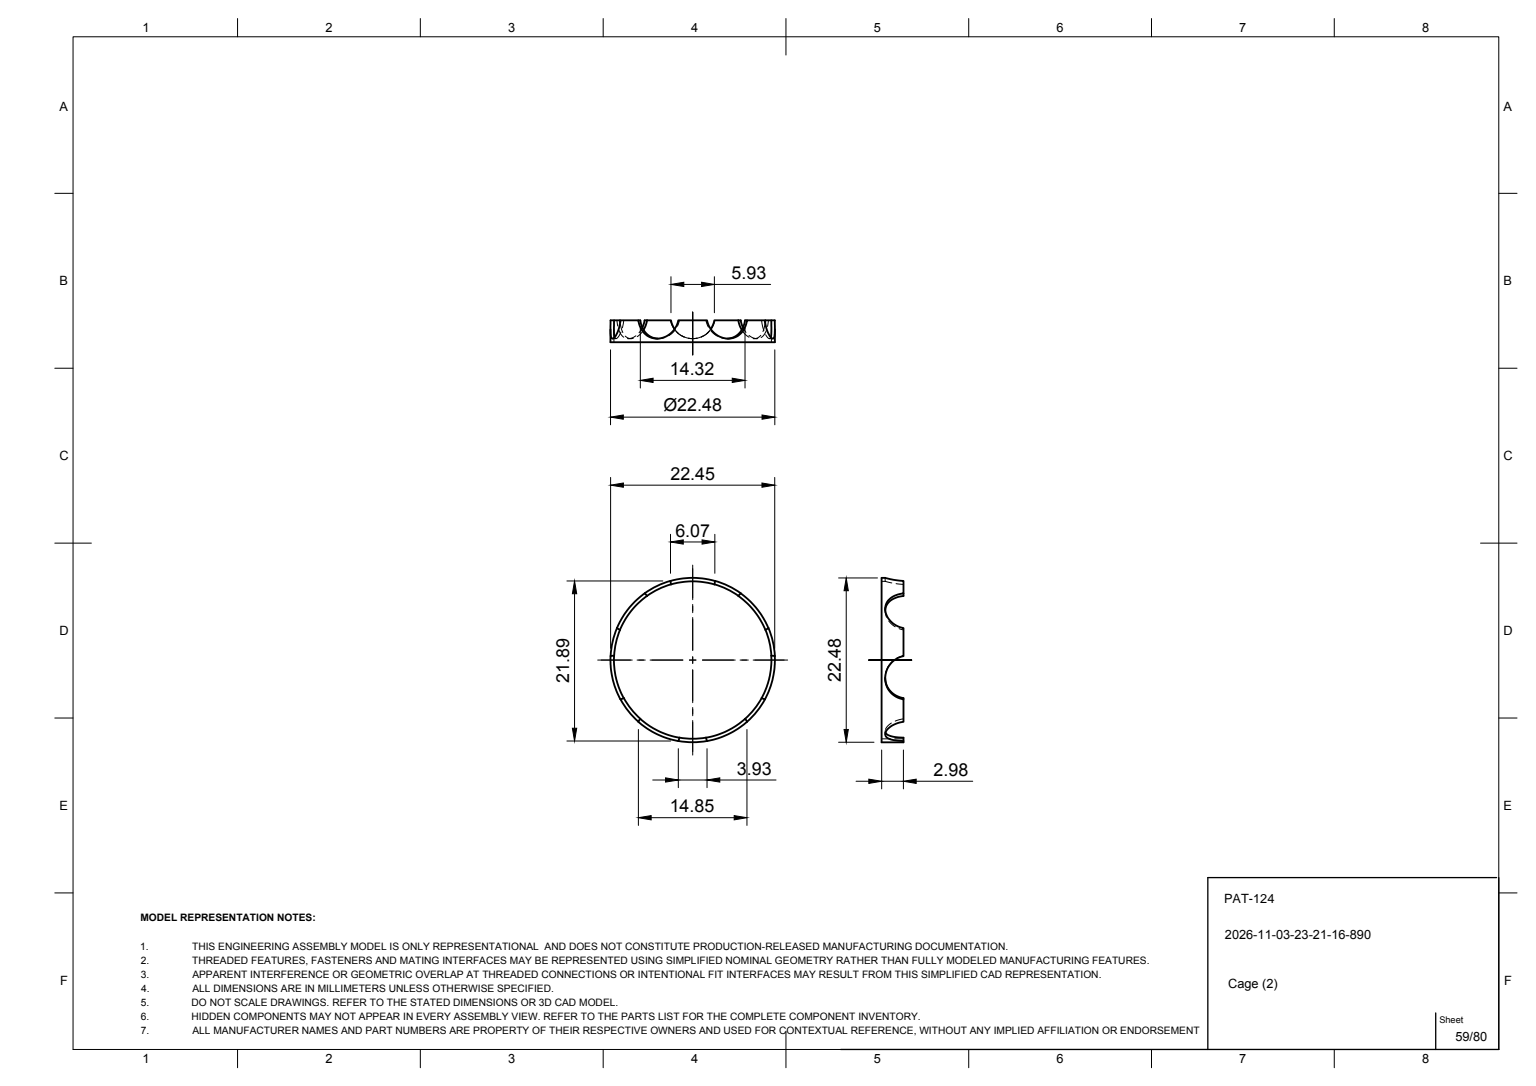
ISO-10303-21;
HEADER;
/* Generated by software containing ST-Developer
 * from STEP Tools, Inc. (www.steptools.com) 
 */

FILE_DESCRIPTION(
/* description */ ('XY cross-slide table'),
/* implementation_level */ '2;1');

FILE_NAME(
/* name */ 'Cage (2).step',
/* time_stamp */ '2026-10-28T03:22:46-07:00',
/* author */ (''),
/* organization */ (''),
/* preprocessor_version */ 'ST-DEVELOPER v20.2',
/* originating_system */ 'Autodesk Translation Framework v15.17.0.0',
/* authorisation */ '');

FILE_SCHEMA (('AUTOMOTIVE_DESIGN { 1 0 10303 214 3 1 1 }'));
ENDSEC;

DATA;
#10=MECHANICAL_DESIGN_GEOMETRIC_PRESENTATION_REPRESENTATION('',(#1745),#62984);
#1037=B_SPLINE_CURVE_WITH_KNOTS('',3,(#48636,#48637,#48638,#48639,#48640,
#48641,#48642,#48643,#48644,#48645,#48646,#48647,#48648,#48649,#48650,#48651,
#48652,#48653,#48654,#48655,#48656,#48657),.UNSPECIFIED.,.F.,.F.,(4,2,2,
2,2,2,2,2,2,2,4),(0.0591825211272536,0.157966726598481,0.236950089897721,
0.315933453196962,0.391576304923761,0.46721915665056,0.54286200837736,0.618504860104159,
0.697488223403399,0.77647158670264,0.875255792173867),.UNSPECIFIED.);
#1038=B_SPLINE_CURVE_WITH_KNOTS('',3,(#48661,#48662,#48663,#48664,#48665,
#48666,#48667,#48668,#48669,#48670,#48671,#48672,#48673,#48674,#48675,#48676,
#48677,#48678,#48679,#48680,#48681,#48682),.UNSPECIFIED.,.F.,.F.,(4,2,2,
2,2,2,2,2,2,2,4),(0.0581119756758434,0.106553146291161,0.213106292582322,
0.30849933801665,0.386091982889075,0.4636846277615,0.541277272633925,0.61886991750635,
0.714262962940678,0.820816109231839,0.869257279847157),.UNSPECIFIED.);
#1039=B_SPLINE_CURVE_WITH_KNOTS('',3,(#48688,#48689,#48690,#48691,#48692,
#48693,#48694,#48695,#48696,#48697,#48698,#48699,#48700,#48701,#48702,#48703,
#48704,#48705,#48706,#48707,#48708,#48709),.UNSPECIFIED.,.F.,.F.,(4,2,2,
2,2,2,2,2,2,2,4),(0.0581119756758434,0.106553146291161,0.213106292582322,
0.30849933801665,0.386091982889075,0.4636846277615,0.541277272633925,0.61886991750635,
0.714262962940679,0.820816109231839,0.869257279847157),.UNSPECIFIED.);
#1040=B_SPLINE_CURVE_WITH_KNOTS('',3,(#48713,#48714,#48715,#48716,#48717,
#48718,#48719,#48720,#48721,#48722,#48723,#48724,#48725,#48726,#48727,#48728,
#48729,#48730,#48731,#48732,#48733,#48734),.UNSPECIFIED.,.F.,.F.,(4,2,2,
2,2,2,2,2,2,2,4),(0.0581119756758433,0.106553146291161,0.213106292582322,
0.308499338016649,0.386091982889075,0.4636846277615,0.541277272633925,0.61886991750635,
0.714262962940678,0.820816109231839,0.869257279847157),.UNSPECIFIED.);
#1041=B_SPLINE_CURVE_WITH_KNOTS('',3,(#48743,#48744,#48745,#48746,#48747,
#48748,#48749,#48750,#48751,#48752,#48753,#48754,#48755,#48756,#48757,#48758,
#48759,#48760,#48761,#48762,#48763,#48764),.UNSPECIFIED.,.F.,.F.,(4,2,2,
2,2,2,2,2,2,2,4),(0.0581119756758433,0.106553146291161,0.213106292582322,
0.30849933801665,0.386091982889075,0.4636846277615,0.541277272633925,0.61886991750635,
0.714262962940678,0.820816109231839,0.869257279847157),.UNSPECIFIED.);
#1042=B_SPLINE_CURVE_WITH_KNOTS('',3,(#48768,#48769,#48770,#48771,#48772,
#48773,#48774,#48775,#48776,#48777,#48778,#48779,#48780,#48781,#48782,#48783,
#48784,#48785,#48786,#48787,#48788,#48789),.UNSPECIFIED.,.F.,.F.,(4,2,2,
2,2,2,2,2,2,2,4),(0.0581119756758434,0.106553146291161,0.213106292582322,
0.30849933801665,0.386091982889075,0.4636846277615,0.541277272633925,0.61886991750635,
0.714262962940678,0.820816109231839,0.869257279847157),.UNSPECIFIED.);
#1043=B_SPLINE_CURVE_WITH_KNOTS('',3,(#48793,#48794,#48795,#48796,#48797,
#48798,#48799,#48800,#48801,#48802,#48803,#48804,#48805,#48806,#48807,#48808,
#48809,#48810,#48811,#48812,#48813,#48814),.UNSPECIFIED.,.F.,.F.,(4,2,2,
2,2,2,2,2,2,2,4),(0.0581119756758434,0.106553146291161,0.213106292582322,
0.30849933801665,0.386091982889075,0.4636846277615,0.541277272633925,0.61886991750635,
0.714262962940678,0.820816109231839,0.869257279847157),.UNSPECIFIED.);
#1044=B_SPLINE_CURVE_WITH_KNOTS('',3,(#48818,#48819,#48820,#48821,#48822,
#48823,#48824,#48825,#48826,#48827,#48828,#48829,#48830,#48831,#48832,#48833,
#48834,#48835,#48836,#48837,#48838,#48839),.UNSPECIFIED.,.F.,.F.,(4,2,2,
2,2,2,2,2,2,2,4),(0.0581119756758433,0.106553146291161,0.213106292582322,
0.30849933801665,0.386091982889075,0.4636846277615,0.541277272633925,0.61886991750635,
0.714262962940678,0.820816109231839,0.869257279847157),.UNSPECIFIED.);
#1045=B_SPLINE_CURVE_WITH_KNOTS('',3,(#48847,#48848,#48849,#48850,#48851,
#48852,#48853,#48854,#48855,#48856,#48857,#48858,#48859,#48860,#48861,#48862,
#48863,#48864,#48865,#48866,#48867,#48868),.UNSPECIFIED.,.F.,.F.,(4,2,2,
2,2,2,2,2,2,2,4),(0.0591825211272536,0.157966726598481,0.236950089897721,
0.315933453196962,0.391576304923761,0.467219156650561,0.54286200837736,
0.618504860104159,0.697488223403399,0.77647158670264,0.875255792173867),
 .UNSPECIFIED.);
#1046=B_SPLINE_CURVE_WITH_KNOTS('',3,(#48876,#48877,#48878,#48879,#48880,
#48881,#48882,#48883,#48884,#48885,#48886,#48887,#48888,#48889,#48890,#48891,
#48892,#48893,#48894,#48895,#48896,#48897),.UNSPECIFIED.,.F.,.F.,(4,2,2,
2,2,2,2,2,2,2,4),(0.0591825211272536,0.157966726598481,0.236950089897722,
0.315933453196962,0.391576304923761,0.467219156650561,0.54286200837736,
0.618504860104159,0.697488223403399,0.77647158670264,0.875255792173867),
 .UNSPECIFIED.);
#1047=B_SPLINE_CURVE_WITH_KNOTS('',3,(#48907,#48908,#48909,#48910,#48911,
#48912,#48913,#48914,#48915,#48916,#48917,#48918,#48919,#48920,#48921,#48922,
#48923,#48924,#48925,#48926,#48927,#48928),.UNSPECIFIED.,.F.,.F.,(4,2,2,
2,2,2,2,2,2,2,4),(0.0591825211272536,0.157966726598481,0.236950089897721,
0.315933453196962,0.391576304923761,0.46721915665056,0.54286200837736,0.618504860104159,
0.697488223403399,0.77647158670264,0.875255792173867),.UNSPECIFIED.);
#1048=B_SPLINE_CURVE_WITH_KNOTS('',3,(#48936,#48937,#48938,#48939,#48940,
#48941,#48942,#48943,#48944,#48945,#48946,#48947,#48948,#48949,#48950,#48951,
#48952,#48953,#48954,#48955,#48956,#48957),.UNSPECIFIED.,.F.,.F.,(4,2,2,
2,2,2,2,2,2,2,4),(0.0591825211272536,0.157966726598481,0.236950089897721,
0.315933453196962,0.391576304923761,0.46721915665056,0.542862008377359,
0.618504860104159,0.697488223403399,0.776471586702639,0.875255792173867),
 .UNSPECIFIED.);
#1049=B_SPLINE_CURVE_WITH_KNOTS('',3,(#48965,#48966,#48967,#48968,#48969,
#48970,#48971,#48972,#48973,#48974,#48975,#48976,#48977,#48978,#48979,#48980,
#48981,#48982,#48983,#48984,#48985,#48986),.UNSPECIFIED.,.F.,.F.,(4,2,2,
2,2,2,2,2,2,2,4),(0.0591825211272536,0.157966726598481,0.236950089897721,
0.315933453196962,0.391576304923761,0.46721915665056,0.54286200837736,0.618504860104159,
0.697488223403399,0.77647158670264,0.875255792173867),.UNSPECIFIED.);
#1050=B_SPLINE_CURVE_WITH_KNOTS('',3,(#48995,#48996,#48997,#48998,#48999,
#49000,#49001,#49002,#49003,#49004,#49005,#49006,#49007,#49008,#49009,#49010,
#49011,#49012,#49013,#49014,#49015,#49016),.UNSPECIFIED.,.F.,.F.,(4,2,2,
2,2,2,2,2,2,2,4),(0.0591825211272536,0.157966726598481,0.236950089897721,
0.315933453196962,0.391576304923761,0.46721915665056,0.542862008377359,
0.618504860104159,0.697488223403399,0.776471586702639,0.875255792173867),
 .UNSPECIFIED.);
#1418=SPHERICAL_SURFACE('',#25587,0.309556);
#1419=SPHERICAL_SURFACE('',#25603,0.309556);
#1420=SPHERICAL_SURFACE('',#25608,0.309556);
#1421=SPHERICAL_SURFACE('',#25614,0.309556);
#1422=SPHERICAL_SURFACE('',#25619,0.309556);
#1423=SPHERICAL_SURFACE('',#25624,0.309556);
#1424=SPHERICAL_SURFACE('',#25632,0.309556);
#1558=SHAPE_REPRESENTATION_RELATIONSHIP('SRR','None',#63414,#1641);
#1641=ADVANCED_BREP_SHAPE_REPRESENTATION('',(#1854),#62951);
#1745=STYLED_ITEM('',(#63912),#1854);
#1854=MANIFOLD_SOLID_BREP('Continuous crown cage',#23043);
#2205=FACE_BOUND('',#5346,.T.);
#2666=PLANE('',#25600);
#2667=PLANE('',#25605);
#2668=PLANE('',#25610);
#2669=PLANE('',#25616);
#2670=PLANE('',#25621);
#2671=PLANE('',#25630);
#2672=PLANE('',#25634);
#2673=PLANE('',#25635);
#3698=FACE_OUTER_BOUND('',#5330,.T.);
#3699=FACE_OUTER_BOUND('',#5331,.T.);
#3700=FACE_OUTER_BOUND('',#5332,.T.);
#3701=FACE_OUTER_BOUND('',#5333,.T.);
#3702=FACE_OUTER_BOUND('',#5334,.T.);
#3703=FACE_OUTER_BOUND('',#5335,.T.);
#3704=FACE_OUTER_BOUND('',#5336,.T.);
#3705=FACE_OUTER_BOUND('',#5337,.T.);
#3706=FACE_OUTER_BOUND('',#5338,.T.);
#3707=FACE_OUTER_BOUND('',#5339,.T.);
#3708=FACE_OUTER_BOUND('',#5340,.T.);
#3709=FACE_OUTER_BOUND('',#5341,.T.);
#3710=FACE_OUTER_BOUND('',#5342,.T.);
#3711=FACE_OUTER_BOUND('',#5343,.T.);
#3712=FACE_OUTER_BOUND('',#5344,.T.);
#3713=FACE_OUTER_BOUND('',#5345,.T.);
#3714=FACE_OUTER_BOUND('',#5347,.T.);
#5330=EDGE_LOOP('',(#18706,#18707,#18708,#18709));
#5331=EDGE_LOOP('',(#18710,#18711,#18712,#18713,#18714,#18715,#18716,#18717,
#18718,#18719,#18720,#18721,#18722,#18723,#18724,#18725,#18726,#18727));
#5332=EDGE_LOOP('',(#18728,#18729,#18730,#18731));
#5333=EDGE_LOOP('',(#18732,#18733,#18734,#18735));
#5334=EDGE_LOOP('',(#18736,#18737,#18738,#18739));
#5335=EDGE_LOOP('',(#18740,#18741,#18742,#18743));
#5336=EDGE_LOOP('',(#18744,#18745,#18746,#18747,#18748,#18749));
#5337=EDGE_LOOP('',(#18750,#18751,#18752,#18753));
#5338=EDGE_LOOP('',(#18754,#18755,#18756,#18757));
#5339=EDGE_LOOP('',(#18758,#18759,#18760,#18761));
#5340=EDGE_LOOP('',(#18762,#18763,#18764,#18765));
#5341=EDGE_LOOP('',(#18766,#18767,#18768,#18769));
#5342=EDGE_LOOP('',(#18770,#18771,#18772,#18773,#18774,#18775,#18776,#18777,
#18778,#18779,#18780,#18781,#18782,#18783,#18784,#18785,#18786,#18787));
#5343=EDGE_LOOP('',(#18788,#18789,#18790,#18791));
#5344=EDGE_LOOP('',(#18792,#18793,#18794,#18795));
#5345=EDGE_LOOP('',(#18796));
#5346=EDGE_LOOP('',(#18797));
#5347=EDGE_LOOP('',(#18798,#18799,#18800,#18801));
#6847=LINE('',#48738,#8334);
#6848=LINE('',#48991,#8335);
#8334=VECTOR('',#30590,1.123812);
#8335=VECTOR('',#30659,1.076188);
#9496=CIRCLE('',#25588,0.303778037777585);
#9497=CIRCLE('',#25589,0.303778037777585);
#9498=CIRCLE('',#25591,1.123812);
#9499=CIRCLE('',#25592,1.123812);
#9500=CIRCLE('',#25593,1.123812);
#9501=CIRCLE('',#25594,1.123812);
#9502=CIRCLE('',#25595,1.123812);
#9503=CIRCLE('',#25596,1.123812);
#9504=CIRCLE('',#25597,1.123812);
#9505=CIRCLE('',#25598,1.123812);
#9506=CIRCLE('',#25599,1.123812);
#9507=CIRCLE('',#25601,1.076188);
#9508=CIRCLE('',#25602,0.303778037777585);
#9509=CIRCLE('',#25604,0.303778037777585);
#9510=CIRCLE('',#25606,1.076188);
#9511=CIRCLE('',#25607,0.303778037777585);
#9512=CIRCLE('',#25609,0.303778037777585);
#9513=CIRCLE('',#25611,1.076188);
#9514=CIRCLE('',#25612,1.076188);
#9515=CIRCLE('',#25613,0.303778037777585);
#9516=CIRCLE('',#25615,0.303778037777585);
#9517=CIRCLE('',#25617,1.076188);
#9518=CIRCLE('',#25618,0.303778037777585);
#9519=CIRCLE('',#25620,0.303778037777585);
#9520=CIRCLE('',#25622,1.076188);
#9521=CIRCLE('',#25623,0.303778037777585);
#9522=CIRCLE('',#25625,0.303778037777585);
#9523=CIRCLE('',#25627,1.076188);
#9524=CIRCLE('',#25628,1.076188);
#9525=CIRCLE('',#25629,1.076188);
#9526=CIRCLE('',#25631,0.303778037777585);
#9527=CIRCLE('',#25633,0.303778037777585);
#11055=VERTEX_POINT('',#48634);
#11056=VERTEX_POINT('',#48635);
#11057=VERTEX_POINT('',#48658);
#11058=VERTEX_POINT('',#48660);
#11059=VERTEX_POINT('',#48685);
#11060=VERTEX_POINT('',#48687);
#11061=VERTEX_POINT('',#48710);
#11062=VERTEX_POINT('',#48712);
#11063=VERTEX_POINT('',#48735);
#11064=VERTEX_POINT('',#48737);
#11065=VERTEX_POINT('',#48740);
#11066=VERTEX_POINT('',#48742);
#11067=VERTEX_POINT('',#48765);
#11068=VERTEX_POINT('',#48767);
#11069=VERTEX_POINT('',#48790);
#11070=VERTEX_POINT('',#48792);
#11071=VERTEX_POINT('',#48815);
#11072=VERTEX_POINT('',#48817);
#11073=VERTEX_POINT('',#48842);
#11074=VERTEX_POINT('',#48846);
#11075=VERTEX_POINT('',#48871);
#11076=VERTEX_POINT('',#48875);
#11077=VERTEX_POINT('',#48900);
#11078=VERTEX_POINT('',#48902);
#11079=VERTEX_POINT('',#48906);
#11080=VERTEX_POINT('',#48931);
#11081=VERTEX_POINT('',#48935);
#11082=VERTEX_POINT('',#48960);
#11083=VERTEX_POINT('',#48964);
#11084=VERTEX_POINT('',#48989);
#11085=VERTEX_POINT('',#48992);
#11086=VERTEX_POINT('',#48994);
#13737=EDGE_CURVE('',#11055,#11056,#1037,.T.);
#13738=EDGE_CURVE('',#11057,#11055,#9496,.T.);
#13739=EDGE_CURVE('',#11058,#11057,#1038,.T.);
#13740=EDGE_CURVE('',#11056,#11058,#9497,.T.);
#13741=EDGE_CURVE('',#11059,#11057,#9498,.T.);
#13742=EDGE_CURVE('',#11059,#11060,#1039,.T.);
#13743=EDGE_CURVE('',#11061,#11060,#9499,.T.);
#13744=EDGE_CURVE('',#11061,#11062,#1040,.T.);
#13745=EDGE_CURVE('',#11063,#11062,#9500,.T.);
#13746=EDGE_CURVE('',#11063,#11064,#6847,.T.);
#13747=EDGE_CURVE('',#11064,#11064,#9501,.T.);
#13748=EDGE_CURVE('',#11065,#11063,#9502,.T.);
#13749=EDGE_CURVE('',#11065,#11066,#1041,.T.);
#13750=EDGE_CURVE('',#11067,#11066,#9503,.T.);
#13751=EDGE_CURVE('',#11067,#11068,#1042,.T.);
#13752=EDGE_CURVE('',#11069,#11068,#9504,.T.);
#13753=EDGE_CURVE('',#11069,#11070,#1043,.T.);
#13754=EDGE_CURVE('',#11071,#11070,#9505,.T.);
#13755=EDGE_CURVE('',#11071,#11072,#1044,.T.);
#13756=EDGE_CURVE('',#11058,#11072,#9506,.T.);
#13757=EDGE_CURVE('',#11055,#11073,#9507,.T.);
#13758=EDGE_CURVE('',#11073,#11059,#9508,.T.);
#13759=EDGE_CURVE('',#11074,#11073,#1045,.T.);
#13760=EDGE_CURVE('',#11060,#11074,#9509,.T.);
#13761=EDGE_CURVE('',#11074,#11075,#9510,.T.);
#13762=EDGE_CURVE('',#11075,#11061,#9511,.T.);
#13763=EDGE_CURVE('',#11076,#11075,#1046,.T.);
#13764=EDGE_CURVE('',#11062,#11076,#9512,.T.);
#13765=EDGE_CURVE('',#11076,#11077,#9513,.T.);
#13766=EDGE_CURVE('',#11077,#11078,#9514,.T.);
#13767=EDGE_CURVE('',#11078,#11065,#9515,.T.);
#13768=EDGE_CURVE('',#11079,#11078,#1047,.T.);
#13769=EDGE_CURVE('',#11066,#11079,#9516,.T.);
#13770=EDGE_CURVE('',#11079,#11080,#9517,.T.);
#13771=EDGE_CURVE('',#11080,#11067,#9518,.T.);
#13772=EDGE_CURVE('',#11081,#11080,#1048,.T.);
#13773=EDGE_CURVE('',#11068,#11081,#9519,.T.);
#13774=EDGE_CURVE('',#11081,#11082,#9520,.T.);
#13775=EDGE_CURVE('',#11082,#11069,#9521,.T.);
#13776=EDGE_CURVE('',#11083,#11082,#1049,.T.);
#13777=EDGE_CURVE('',#11070,#11083,#9522,.T.);
#13778=EDGE_CURVE('',#11084,#11084,#9523,.T.);
#13779=EDGE_CURVE('',#11084,#11077,#6848,.T.);
#13780=EDGE_CURVE('',#11085,#11056,#9524,.T.);
#13781=EDGE_CURVE('',#11085,#11086,#1050,.T.);
#13782=EDGE_CURVE('',#11083,#11086,#9525,.T.);
#13783=EDGE_CURVE('',#11072,#11085,#9526,.T.);
#13784=EDGE_CURVE('',#11086,#11071,#9527,.T.);
#18706=ORIENTED_EDGE('',*,*,#13737,.F.);
#18707=ORIENTED_EDGE('',*,*,#13738,.F.);
#18708=ORIENTED_EDGE('',*,*,#13739,.F.);
#18709=ORIENTED_EDGE('',*,*,#13740,.F.);
#18710=ORIENTED_EDGE('',*,*,#13739,.T.);
#18711=ORIENTED_EDGE('',*,*,#13741,.F.);
#18712=ORIENTED_EDGE('',*,*,#13742,.T.);
#18713=ORIENTED_EDGE('',*,*,#13743,.F.);
#18714=ORIENTED_EDGE('',*,*,#13744,.T.);
#18715=ORIENTED_EDGE('',*,*,#13745,.F.);
#18716=ORIENTED_EDGE('',*,*,#13746,.T.);
#18717=ORIENTED_EDGE('',*,*,#13747,.F.);
#18718=ORIENTED_EDGE('',*,*,#13746,.F.);
#18719=ORIENTED_EDGE('',*,*,#13748,.F.);
#18720=ORIENTED_EDGE('',*,*,#13749,.T.);
#18721=ORIENTED_EDGE('',*,*,#13750,.F.);
#18722=ORIENTED_EDGE('',*,*,#13751,.T.);
#18723=ORIENTED_EDGE('',*,*,#13752,.F.);
#18724=ORIENTED_EDGE('',*,*,#13753,.T.);
#18725=ORIENTED_EDGE('',*,*,#13754,.F.);
#18726=ORIENTED_EDGE('',*,*,#13755,.T.);
#18727=ORIENTED_EDGE('',*,*,#13756,.F.);
#18728=ORIENTED_EDGE('',*,*,#13738,.T.);
#18729=ORIENTED_EDGE('',*,*,#13757,.T.);
#18730=ORIENTED_EDGE('',*,*,#13758,.T.);
#18731=ORIENTED_EDGE('',*,*,#13741,.T.);
#18732=ORIENTED_EDGE('',*,*,#13759,.F.);
#18733=ORIENTED_EDGE('',*,*,#13760,.F.);
#18734=ORIENTED_EDGE('',*,*,#13742,.F.);
#18735=ORIENTED_EDGE('',*,*,#13758,.F.);
#18736=ORIENTED_EDGE('',*,*,#13760,.T.);
#18737=ORIENTED_EDGE('',*,*,#13761,.T.);
#18738=ORIENTED_EDGE('',*,*,#13762,.T.);
#18739=ORIENTED_EDGE('',*,*,#13743,.T.);
#18740=ORIENTED_EDGE('',*,*,#13763,.F.);
#18741=ORIENTED_EDGE('',*,*,#13764,.F.);
#18742=ORIENTED_EDGE('',*,*,#13744,.F.);
#18743=ORIENTED_EDGE('',*,*,#13762,.F.);
#18744=ORIENTED_EDGE('',*,*,#13764,.T.);
#18745=ORIENTED_EDGE('',*,*,#13765,.T.);
#18746=ORIENTED_EDGE('',*,*,#13766,.T.);
#18747=ORIENTED_EDGE('',*,*,#13767,.T.);
#18748=ORIENTED_EDGE('',*,*,#13748,.T.);
#18749=ORIENTED_EDGE('',*,*,#13745,.T.);
#18750=ORIENTED_EDGE('',*,*,#13768,.F.);
#18751=ORIENTED_EDGE('',*,*,#13769,.F.);
#18752=ORIENTED_EDGE('',*,*,#13749,.F.);
#18753=ORIENTED_EDGE('',*,*,#13767,.F.);
#18754=ORIENTED_EDGE('',*,*,#13769,.T.);
#18755=ORIENTED_EDGE('',*,*,#13770,.T.);
#18756=ORIENTED_EDGE('',*,*,#13771,.T.);
#18757=ORIENTED_EDGE('',*,*,#13750,.T.);
#18758=ORIENTED_EDGE('',*,*,#13772,.F.);
#18759=ORIENTED_EDGE('',*,*,#13773,.F.);
#18760=ORIENTED_EDGE('',*,*,#13751,.F.);
#18761=ORIENTED_EDGE('',*,*,#13771,.F.);
#18762=ORIENTED_EDGE('',*,*,#13773,.T.);
#18763=ORIENTED_EDGE('',*,*,#13774,.T.);
#18764=ORIENTED_EDGE('',*,*,#13775,.T.);
#18765=ORIENTED_EDGE('',*,*,#13752,.T.);
#18766=ORIENTED_EDGE('',*,*,#13753,.F.);
#18767=ORIENTED_EDGE('',*,*,#13775,.F.);
#18768=ORIENTED_EDGE('',*,*,#13776,.F.);
#18769=ORIENTED_EDGE('',*,*,#13777,.F.);
#18770=ORIENTED_EDGE('',*,*,#13778,.F.);
#18771=ORIENTED_EDGE('',*,*,#13779,.T.);
#18772=ORIENTED_EDGE('',*,*,#13765,.F.);
#18773=ORIENTED_EDGE('',*,*,#13763,.T.);
#18774=ORIENTED_EDGE('',*,*,#13761,.F.);
#18775=ORIENTED_EDGE('',*,*,#13759,.T.);
#18776=ORIENTED_EDGE('',*,*,#13757,.F.);
#18777=ORIENTED_EDGE('',*,*,#13737,.T.);
#18778=ORIENTED_EDGE('',*,*,#13780,.F.);
#18779=ORIENTED_EDGE('',*,*,#13781,.T.);
#18780=ORIENTED_EDGE('',*,*,#13782,.F.);
#18781=ORIENTED_EDGE('',*,*,#13776,.T.);
#18782=ORIENTED_EDGE('',*,*,#13774,.F.);
#18783=ORIENTED_EDGE('',*,*,#13772,.T.);
#18784=ORIENTED_EDGE('',*,*,#13770,.F.);
#18785=ORIENTED_EDGE('',*,*,#13768,.T.);
#18786=ORIENTED_EDGE('',*,*,#13766,.F.);
#18787=ORIENTED_EDGE('',*,*,#13779,.F.);
#18788=ORIENTED_EDGE('',*,*,#13740,.T.);
#18789=ORIENTED_EDGE('',*,*,#13756,.T.);
#18790=ORIENTED_EDGE('',*,*,#13783,.T.);
#18791=ORIENTED_EDGE('',*,*,#13780,.T.);
#18792=ORIENTED_EDGE('',*,*,#13755,.F.);
#18793=ORIENTED_EDGE('',*,*,#13784,.F.);
#18794=ORIENTED_EDGE('',*,*,#13781,.F.);
#18795=ORIENTED_EDGE('',*,*,#13783,.F.);
#18796=ORIENTED_EDGE('',*,*,#13747,.T.);
#18797=ORIENTED_EDGE('',*,*,#13778,.T.);
#18798=ORIENTED_EDGE('',*,*,#13777,.T.);
#18799=ORIENTED_EDGE('',*,*,#13782,.T.);
#18800=ORIENTED_EDGE('',*,*,#13784,.T.);
#18801=ORIENTED_EDGE('',*,*,#13754,.T.);
#21422=CYLINDRICAL_SURFACE('',#25590,1.123812);
#21423=CYLINDRICAL_SURFACE('',#25626,1.076188);
#22479=ADVANCED_FACE('',(#3698),#1418,.F.);
#22480=ADVANCED_FACE('',(#3699),#21422,.T.);
#22481=ADVANCED_FACE('',(#3700),#2666,.T.);
#22482=ADVANCED_FACE('',(#3701),#1419,.F.);
#22483=ADVANCED_FACE('',(#3702),#2667,.T.);
#22484=ADVANCED_FACE('',(#3703),#1420,.F.);
#22485=ADVANCED_FACE('',(#3704),#2668,.T.);
#22486=ADVANCED_FACE('',(#3705),#1421,.F.);
#22487=ADVANCED_FACE('',(#3706),#2669,.T.);
#22488=ADVANCED_FACE('',(#3707),#1422,.F.);
#22489=ADVANCED_FACE('',(#3708),#2670,.T.);
#22490=ADVANCED_FACE('',(#3709),#1423,.F.);
#22491=ADVANCED_FACE('',(#3710),#21423,.F.);
#22492=ADVANCED_FACE('',(#3711),#2671,.T.);
#22493=ADVANCED_FACE('',(#3712),#1424,.F.);
#22494=ADVANCED_FACE('',(#3713,#2205),#2672,.T.);
#22495=ADVANCED_FACE('',(#3714),#2673,.T.);
#23043=CLOSED_SHELL('',(#22479,#22480,#22481,#22482,#22483,#22484,#22485,
#22486,#22487,#22488,#22489,#22490,#22491,#22492,#22493,#22494,#22495));
#25586=AXIS2_PLACEMENT_3D('',#48632,#30574,#30575);
#25587=AXIS2_PLACEMENT_3D('',#48633,#30576,#30577);
#25588=AXIS2_PLACEMENT_3D('',#48659,#30578,#30579);
#25589=AXIS2_PLACEMENT_3D('',#48683,#30580,#30581);
#25590=AXIS2_PLACEMENT_3D('',#48684,#30582,#30583);
#25591=AXIS2_PLACEMENT_3D('',#48686,#30584,#30585);
#25592=AXIS2_PLACEMENT_3D('',#48711,#30586,#30587);
#25593=AXIS2_PLACEMENT_3D('',#48736,#30588,#30589);
#25594=AXIS2_PLACEMENT_3D('',#48739,#30591,#30592);
#25595=AXIS2_PLACEMENT_3D('',#48741,#30593,#30594);
#25596=AXIS2_PLACEMENT_3D('',#48766,#30595,#30596);
#25597=AXIS2_PLACEMENT_3D('',#48791,#30597,#30598);
#25598=AXIS2_PLACEMENT_3D('',#48816,#30599,#30600);
#25599=AXIS2_PLACEMENT_3D('',#48840,#30601,#30602);
#25600=AXIS2_PLACEMENT_3D('',#48841,#30603,#30604);
#25601=AXIS2_PLACEMENT_3D('',#48843,#30605,#30606);
#25602=AXIS2_PLACEMENT_3D('',#48844,#30607,#30608);
#25603=AXIS2_PLACEMENT_3D('',#48845,#30609,#30610);
#25604=AXIS2_PLACEMENT_3D('',#48869,#30611,#30612);
#25605=AXIS2_PLACEMENT_3D('',#48870,#30613,#30614);
#25606=AXIS2_PLACEMENT_3D('',#48872,#30615,#30616);
#25607=AXIS2_PLACEMENT_3D('',#48873,#30617,#30618);
#25608=AXIS2_PLACEMENT_3D('',#48874,#30619,#30620);
#25609=AXIS2_PLACEMENT_3D('',#48898,#30621,#30622);
#25610=AXIS2_PLACEMENT_3D('',#48899,#30623,#30624);
#25611=AXIS2_PLACEMENT_3D('',#48901,#30625,#30626);
#25612=AXIS2_PLACEMENT_3D('',#48903,#30627,#30628);
#25613=AXIS2_PLACEMENT_3D('',#48904,#30629,#30630);
#25614=AXIS2_PLACEMENT_3D('',#48905,#30631,#30632);
#25615=AXIS2_PLACEMENT_3D('',#48929,#30633,#30634);
#25616=AXIS2_PLACEMENT_3D('',#48930,#30635,#30636);
#25617=AXIS2_PLACEMENT_3D('',#48932,#30637,#30638);
#25618=AXIS2_PLACEMENT_3D('',#48933,#30639,#30640);
#25619=AXIS2_PLACEMENT_3D('',#48934,#30641,#30642);
#25620=AXIS2_PLACEMENT_3D('',#48958,#30643,#30644);
#25621=AXIS2_PLACEMENT_3D('',#48959,#30645,#30646);
#25622=AXIS2_PLACEMENT_3D('',#48961,#30647,#30648);
#25623=AXIS2_PLACEMENT_3D('',#48962,#30649,#30650);
#25624=AXIS2_PLACEMENT_3D('',#48963,#30651,#30652);
#25625=AXIS2_PLACEMENT_3D('',#48987,#30653,#30654);
#25626=AXIS2_PLACEMENT_3D('',#48988,#30655,#30656);
#25627=AXIS2_PLACEMENT_3D('',#48990,#30657,#30658);
#25628=AXIS2_PLACEMENT_3D('',#48993,#30660,#30661);
#25629=AXIS2_PLACEMENT_3D('',#49017,#30662,#30663);
#25630=AXIS2_PLACEMENT_3D('',#49018,#30664,#30665);
#25631=AXIS2_PLACEMENT_3D('',#49019,#30666,#30667);
#25632=AXIS2_PLACEMENT_3D('',#49020,#30668,#30669);
#25633=AXIS2_PLACEMENT_3D('',#49021,#30670,#30671);
#25634=AXIS2_PLACEMENT_3D('',#49022,#30672,#30673);
#25635=AXIS2_PLACEMENT_3D('',#49023,#30674,#30675);
#30574=DIRECTION('axis',(0.,0.,1.));
#30575=DIRECTION('refdir',(1.,0.,0.));
#30576=DIRECTION('center_axis',(0.,0.,1.));
#30577=DIRECTION('ref_axis',(1.,0.,0.));
#30578=DIRECTION('center_axis',(0.,-1.,0.));
#30579=DIRECTION('ref_axis',(0.,0.,-1.));
#30580=DIRECTION('center_axis',(0.,-1.,0.));
#30581=DIRECTION('ref_axis',(0.,0.,-1.));
#30582=DIRECTION('center_axis',(0.,1.,0.));
#30583=DIRECTION('ref_axis',(1.,0.,0.));
#30584=DIRECTION('center_axis',(0.,1.,0.));
#30585=DIRECTION('ref_axis',(1.,0.,0.));
#30586=DIRECTION('center_axis',(0.,1.,0.));
#30587=DIRECTION('ref_axis',(1.,0.,0.));
#30588=DIRECTION('center_axis',(0.,1.,0.));
#30589=DIRECTION('ref_axis',(1.,0.,0.));
#30590=DIRECTION('',(0.,-1.,0.));
#30591=DIRECTION('center_axis',(0.,-1.,0.));
#30592=DIRECTION('ref_axis',(1.,0.,0.));
#30593=DIRECTION('center_axis',(0.,1.,0.));
#30594=DIRECTION('ref_axis',(1.,0.,0.));
#30595=DIRECTION('center_axis',(0.,1.,0.));
#30596=DIRECTION('ref_axis',(1.,0.,0.));
#30597=DIRECTION('center_axis',(0.,1.,0.));
#30598=DIRECTION('ref_axis',(1.,0.,0.));
#30599=DIRECTION('center_axis',(0.,1.,0.));
#30600=DIRECTION('ref_axis',(1.,0.,0.));
#30601=DIRECTION('center_axis',(0.,1.,0.));
#30602=DIRECTION('ref_axis',(1.,0.,0.));
#30603=DIRECTION('center_axis',(0.,1.,0.));
#30604=DIRECTION('ref_axis',(1.,0.,0.));
#30605=DIRECTION('center_axis',(0.,-1.,0.));
#30606=DIRECTION('ref_axis',(1.,0.,0.));
#30607=DIRECTION('center_axis',(0.,-1.,0.));
#30608=DIRECTION('ref_axis',(0.,0.,-1.));
#30609=DIRECTION('center_axis',(8.96625347776458E-17,0.,1.));
#30610=DIRECTION('ref_axis',(1.,0.,0.));
#30611=DIRECTION('center_axis',(0.,-1.,0.));
#30612=DIRECTION('ref_axis',(0.,0.,-1.));
#30613=DIRECTION('center_axis',(0.,1.,0.));
#30614=DIRECTION('ref_axis',(1.,0.,0.));
#30615=DIRECTION('center_axis',(0.,-1.,0.));
#30616=DIRECTION('ref_axis',(1.,0.,0.));
#30617=DIRECTION('center_axis',(0.,-1.,0.));
#30618=DIRECTION('ref_axis',(0.,0.,-1.));
#30619=DIRECTION('center_axis',(0.,0.,1.));
#30620=DIRECTION('ref_axis',(1.,0.,0.));
#30621=DIRECTION('center_axis',(0.,-1.,0.));
#30622=DIRECTION('ref_axis',(0.,0.,-1.));
#30623=DIRECTION('center_axis',(0.,1.,0.));
#30624=DIRECTION('ref_axis',(1.,0.,0.));
#30625=DIRECTION('center_axis',(0.,-1.,0.));
#30626=DIRECTION('ref_axis',(1.,0.,0.));
#30627=DIRECTION('center_axis',(0.,-1.,0.));
#30628=DIRECTION('ref_axis',(1.,0.,0.));
#30629=DIRECTION('center_axis',(0.,-1.,0.));
#30630=DIRECTION('ref_axis',(0.,0.,-1.));
#30631=DIRECTION('center_axis',(0.,0.,1.));
#30632=DIRECTION('ref_axis',(1.,0.,0.));
#30633=DIRECTION('center_axis',(0.,-1.,0.));
#30634=DIRECTION('ref_axis',(0.,0.,-1.));
#30635=DIRECTION('center_axis',(0.,1.,0.));
#30636=DIRECTION('ref_axis',(1.,0.,0.));
#30637=DIRECTION('center_axis',(0.,-1.,0.));
#30638=DIRECTION('ref_axis',(1.,0.,0.));
#30639=DIRECTION('center_axis',(0.,-1.,0.));
#30640=DIRECTION('ref_axis',(0.,0.,-1.));
#30641=DIRECTION('center_axis',(8.96625347776458E-17,0.,1.));
#30642=DIRECTION('ref_axis',(1.,0.,0.));
#30643=DIRECTION('center_axis',(0.,-1.,0.));
#30644=DIRECTION('ref_axis',(0.,0.,-1.));
#30645=DIRECTION('center_axis',(0.,1.,0.));
#30646=DIRECTION('ref_axis',(1.,0.,0.));
#30647=DIRECTION('center_axis',(0.,-1.,0.));
#30648=DIRECTION('ref_axis',(1.,0.,0.));
#30649=DIRECTION('center_axis',(0.,-1.,0.));
#30650=DIRECTION('ref_axis',(0.,0.,-1.));
#30651=DIRECTION('center_axis',(0.,0.,1.));
#30652=DIRECTION('ref_axis',(1.,0.,0.));
#30653=DIRECTION('center_axis',(0.,-1.,0.));
#30654=DIRECTION('ref_axis',(0.,0.,-1.));
#30655=DIRECTION('center_axis',(0.,1.,0.));
#30656=DIRECTION('ref_axis',(1.,0.,0.));
#30657=DIRECTION('center_axis',(0.,1.,0.));
#30658=DIRECTION('ref_axis',(1.,0.,0.));
#30659=DIRECTION('',(0.,1.,0.));
#30660=DIRECTION('center_axis',(0.,-1.,0.));
#30661=DIRECTION('ref_axis',(1.,0.,0.));
#30662=DIRECTION('center_axis',(0.,-1.,0.));
#30663=DIRECTION('ref_axis',(1.,0.,0.));
#30664=DIRECTION('center_axis',(0.,1.,0.));
#30665=DIRECTION('ref_axis',(1.,0.,0.));
#30666=DIRECTION('center_axis',(0.,-1.,0.));
#30667=DIRECTION('ref_axis',(0.,0.,-1.));
#30668=DIRECTION('center_axis',(0.,0.,1.));
#30669=DIRECTION('ref_axis',(1.,0.,0.));
#30670=DIRECTION('center_axis',(0.,-1.,0.));
#30671=DIRECTION('ref_axis',(0.,0.,-1.));
#30672=DIRECTION('center_axis',(0.,-1.,0.));
#30673=DIRECTION('ref_axis',(-1.,0.,0.));
#30674=DIRECTION('center_axis',(0.,1.,0.));
#30675=DIRECTION('ref_axis',(1.,0.,0.));
#48632=CARTESIAN_POINT('',(0.,0.,0.));
#48633=CARTESIAN_POINT('Origin',(0.685838782044607,0.,0.860014630714833));
#48634=CARTESIAN_POINT('',(0.413083465285518,-0.05953,0.993751811093549));
#48635=CARTESIAN_POINT('',(0.876916659919095,-0.05953,0.623857181492959));
#48636=CARTESIAN_POINT('Ctrl Pts',(0.413083465285518,-0.05953,0.993751811093549));
#48637=CARTESIAN_POINT('Ctrl Pts',(0.419070565453383,-0.0925528133349865,
0.991263089003441));
#48638=CARTESIAN_POINT('Ctrl Pts',(0.430199341854858,-0.124911173756694,
0.986608710139579));
#48639=CARTESIAN_POINT('Ctrl Pts',(0.457978755888596,-0.177924977804098,
0.973971221090534));
#48640=CARTESIAN_POINT('Ctrl Pts',(0.473077587363685,-0.199697230012983,
0.966820759530997));
#48641=CARTESIAN_POINT('Ctrl Pts',(0.507057380724533,-0.237895043532788,
0.949440676105255));
#48642=CARTESIAN_POINT('Ctrl Pts',(0.525933334162555,-0.254319232363049,
0.939198248544428));
#48643=CARTESIAN_POINT('Ctrl Pts',(0.564362943424238,-0.28018331644634,
0.916597376014514));
#48644=CARTESIAN_POINT('Ctrl Pts',(0.585840553788742,-0.29104845371857,
0.903141581680914));
#48645=CARTESIAN_POINT('Ctrl Pts',(0.629305439856167,-0.30527573347708,
0.873412008702649));
#48646=CARTESIAN_POINT('Ctrl Pts',(0.651278921914856,-0.308638795020976,
0.857118508332695));
#48647=CARTESIAN_POINT('Ctrl Pts',(0.690705563850638,-0.308638795020976,
0.825676810575914));
#48648=CARTESIAN_POINT('Ctrl Pts',(0.711480111898423,-0.30527573347708,
0.807879894508811));
#48649=CARTESIAN_POINT('Ctrl Pts',(0.750136149454208,-0.29104845371857,
0.772120216227122));
#48650=CARTESIAN_POINT('Ctrl Pts',(0.768033796848072,-0.28018331644634,
0.754175290318038));
#48651=CARTESIAN_POINT('Ctrl Pts',(0.798619410861634,-0.254319232363049,
0.721738358858166));
#48652=CARTESIAN_POINT('Ctrl Pts',(0.812805334167529,-0.237895043532788,
0.705614819529209));
#48653=CARTESIAN_POINT('Ctrl Pts',(0.837310877969633,-0.199697230012983,
0.676354402927683));
#48654=CARTESIAN_POINT('Ctrl Pts',(0.847641868610495,-0.177924977804098,
0.663225258065736));
#48655=CARTESIAN_POINT('Ctrl Pts',(0.866144010579847,-0.124911173756694,
0.638954437806245));
#48656=CARTESIAN_POINT('Ctrl Pts',(0.873158080166742,-0.0925528133349865,
0.62914037979579));
#48657=CARTESIAN_POINT('Ctrl Pts',(0.876916659919095,-0.05953,0.623857181492959));
#48658=CARTESIAN_POINT('',(0.437601487681057,-0.05953,1.03511272300331));
#48659=CARTESIAN_POINT('Origin',(0.685838782044607,-0.05953,0.860014630714833));
#48660=CARTESIAN_POINT('',(0.911784794170997,-0.05953,0.656964154625313));
#48661=CARTESIAN_POINT('Ctrl Pts',(0.911784794170998,-0.0595300000000001,
0.656964154625312));
#48662=CARTESIAN_POINT('Ctrl Pts',(0.909827729890942,-0.0762225747374255,
0.659680317203144));
#48663=CARTESIAN_POINT('Ctrl Pts',(0.907004864562642,-0.0928409665394228,
0.663576540841106));
#48664=CARTESIAN_POINT('Ctrl Pts',(0.895234408667242,-0.144299303100741,
0.679480524217551));
#48665=CARTESIAN_POINT('Ctrl Pts',(0.882797231409153,-0.177024326825049,
0.695831250979106));
#48666=CARTESIAN_POINT('Ctrl Pts',(0.854332839576145,-0.227269801620064,
0.73042219438957));
#48667=CARTESIAN_POINT('Ctrl Pts',(0.834863020612702,-0.251265615809407,
0.752807465209441));
#48668=CARTESIAN_POINT('Ctrl Pts',(0.800439809856111,-0.279889827963178,
0.789147407129766));
#48669=CARTESIAN_POINT('Ctrl Pts',(0.781998747691871,-0.290879136862659,
0.80756613568454));
#48670=CARTESIAN_POINT('Ctrl Pts',(0.742239891936898,-0.305251990234487,
0.844254137480382));
#48671=CARTESIAN_POINT('Ctrl Pts',(0.720906778729541,-0.308638795020976,
0.862505527716294));
#48672=CARTESIAN_POINT('Ctrl Pts',(0.680463863683392,-0.308638795020976,
0.894757676234429));
#48673=CARTESIAN_POINT('Ctrl Pts',(0.657923009631182,-0.305251990234488,
0.91149460735272));
#48674=CARTESIAN_POINT('Ctrl Pts',(0.613307674922609,-0.290879136862659,
0.942092777160053));
#48675=CARTESIAN_POINT('Ctrl Pts',(0.591247219971725,-0.279889827963178,
0.955972930713954));
#48676=CARTESIAN_POINT('Ctrl Pts',(0.548158511259202,-0.251265615809407,
0.981446681891443));
#48677=CARTESIAN_POINT('Ctrl Pts',(0.522002043615455,-0.227269801620063,
0.995447160474328));
#48678=CARTESIAN_POINT('Ctrl Pts',(0.481944444320713,-0.177024326825049,
1.01550068154148));
#48679=CARTESIAN_POINT('Ctrl Pts',(0.463236132117164,-0.14429930310074,
1.0239876538093));
#48680=CARTESIAN_POINT('Ctrl Pts',(0.445111721969657,-0.0928409665394226,
1.03192403056628));
#48681=CARTESIAN_POINT('Ctrl Pts',(0.440685038163619,-0.0762225747374254,
1.03380912944435));
#48682=CARTESIAN_POINT('Ctrl Pts',(0.437601487681056,-0.05953,1.03511272300331));
#48683=CARTESIAN_POINT('Origin',(0.685838782044607,-0.05953,0.860014630714833));
#48684=CARTESIAN_POINT('Origin',(0.,-0.208355,0.));
#48685=CARTESIAN_POINT('',(0.0548532617164168,-0.05953,1.12247250791415));
#48686=CARTESIAN_POINT('Origin',(0.,-0.05953,0.));
#48687=CARTESIAN_POINT('',(-0.536443649899848,-0.05953,0.987512846410683));
#48688=CARTESIAN_POINT('Ctrl Pts',(0.0548532617164173,-0.0595300000000001,
1.12247250791414));
#48689=CARTESIAN_POINT('Ctrl Pts',(0.05150947068137,-0.0762225747374254,
1.12263591311425));
#48690=CARTESIAN_POINT('Ctrl Pts',(0.0467032526342597,-0.0928409665394227,
1.12285816383385));
#48691=CARTESIAN_POINT('Ctrl Pts',(0.0269302585198975,-0.144299303100741,
1.12357162229597));
#48692=CARTESIAN_POINT('Ctrl Pts',(0.006392292392153,-0.177024326825049,
1.12404235695137));
#48693=CARTESIAN_POINT('Ctrl Pts',(-0.0383992541984087,-0.227269801620063,
1.12335509974011));
#48694=CARTESIAN_POINT('Ctrl Pts',(-0.0680399972366993,-0.251265615809407,
1.12208997038458));
#48695=CARTESIAN_POINT('Ctrl Pts',(-0.117914228755037,-0.279889827963178,
1.1178344036749));
#48696=CARTESIAN_POINT('Ctrl Pts',(-0.14381238480104,-0.290879136862659,
1.11490049012186));
#48697=CARTESIAN_POINT('Ctrl Pts',(-0.19728546073067,-0.305251990234488,
1.10669035995599));
#48698=CARTESIAN_POINT('Ctrl Pts',(-0.224855950742601,-0.308638795020976,
1.10139101611326));
#48699=CARTESIAN_POINT('Ctrl Pts',(-0.275287440920027,-0.308638795020976,
1.0898803575765));
#48700=CARTESIAN_POINT('Ctrl Pts',(-0.302426893214945,-0.305251990234488,
1.08269251410343));
#48701=CARTESIAN_POINT('Ctrl Pts',(-0.35416671187353,-0.290879136862659,
1.06688848765783));
#48702=CARTESIAN_POINT('Ctrl Pts',(-0.3787731215897,-0.279889827963178,
1.05829506364875));
#48703=CARTESIAN_POINT('Ctrl Pts',(-0.425554672694338,-0.251265615809407,
1.04048957871266));
#48704=CARTESIAN_POINT('Ctrl Pts',(-0.452808978448581,-0.227269801620063,
1.02876878445619));
#48705=CARTESIAN_POINT('Ctrl Pts',(-0.493462957200432,-0.177024326825049,
1.0099536580922));
#48706=CARTESIAN_POINT('Ctrl Pts',(-0.511762781179148,-0.14429930310074,
1.00061845128527));
#48707=CARTESIAN_POINT('Ctrl Pts',(-0.529268075276157,-0.0928409665394226,
0.991396466802468));
#48708=CARTESIAN_POINT('Ctrl Pts',(-0.533501897135713,-0.0762225747374254,
0.989110885965947));
#48709=CARTESIAN_POINT('Ctrl Pts',(-0.536443649899848,-0.0595300000000001,
0.987512846410683));
#48710=CARTESIAN_POINT('',(-0.843383895613249,-0.05953,0.742736168477219));
#48711=CARTESIAN_POINT('Origin',(0.,-0.05953,0.));
#48712=CARTESIAN_POINT('',(-1.10653577764992,-0.05953,0.196295654879792));
#48713=CARTESIAN_POINT('Ctrl Pts',(-0.843383895613249,-0.0595300000000001,
0.742736168477219));
#48714=CARTESIAN_POINT('Ctrl Pts',(-0.84559647055299,-0.0762225747374255,
0.740223768851062));
#48715=CARTESIAN_POINT('Ctrl Pts',(-0.848766861100456,-0.0928409665394227,
0.736604687327351));
#48716=CARTESIAN_POINT('Ctrl Pts',(-0.861652925570091,-0.144299303100741,
0.721590372101268));
#48717=CARTESIAN_POINT('Ctrl Pts',(-0.87482617317514,-0.177024326825049,
0.705826641853758));
#48718=CARTESIAN_POINT('Ctrl Pts',(-0.902215926359523,-0.227269801620063,
0.670378702718353));
#48719=CARTESIAN_POINT('Ctrl Pts',(-0.919707509403859,-0.251265615809407,
0.646415841396062));
#48720=CARTESIAN_POINT('Ctrl Pts',(-0.947476448101718,-0.279889827963178,
0.604769294586516));
#48721=CARTESIAN_POINT('Ctrl Pts',(-0.961329858300736,-0.290879136862659,
0.582692035672022));
#48722=CARTESIAN_POINT('Ctrl Pts',(-0.988250837578047,-0.305251990234488,
0.535766169015486));
#48723=CARTESIAN_POINT('Ctrl Pts',(-1.00129756308006,-0.308638795020976,
0.510906605094603));
#48724=CARTESIAN_POINT('Ctrl Pts',(-1.02374168767024,-0.308638795020976,
0.46430090015576));
#48725=CARTESIAN_POINT('Ctrl Pts',(-1.03504317708586,-0.305251990234488,
0.438600874831839));
#48726=CARTESIAN_POINT('Ctrl Pts',(-1.05494634094458,-0.290879136862659,
0.388295406390235));
#48727=CARTESIAN_POINT('Ctrl Pts',(-1.06356957703048,-0.279889827963178,
0.363699428370917));
#48728=CARTESIAN_POINT('Ctrl Pts',(-1.0788165083757,-0.251265615809407,
0.316022600643821));
#48729=CARTESIAN_POINT('Ctrl Pts',(-1.08664560412098,-0.227269801620063,
0.287406530683752));
#48730=CARTESIAN_POINT('Ctrl Pts',(-1.09728268713976,-0.177024326825049,
0.243890930799337));
#48731=CARTESIAN_POINT('Ctrl Pts',(-1.10139388218929,-0.144299303100741,
0.22376314604679));
#48732=CARTESIAN_POINT('Ctrl Pts',(-1.10509821673782,-0.0928409665394227,
0.204327142733961));
#48733=CARTESIAN_POINT('Ctrl Pts',(-1.10595102243643,-0.0762225747374254,
0.199591971170104));
#48734=CARTESIAN_POINT('Ctrl Pts',(-1.10653577764992,-0.0595300000000001,
0.196295654879792));
#48735=CARTESIAN_POINT('',(-1.123812,-0.05953,1.37627276864339E-16));
#48736=CARTESIAN_POINT('Origin',(0.,-0.05953,0.));
#48737=CARTESIAN_POINT('',(-1.123812,-0.35718,1.37627276864339E-16));
#48738=CARTESIAN_POINT('',(-1.123812,-0.208355,1.37627276864339E-16));
#48739=CARTESIAN_POINT('Origin',(0.,-0.35718,0.));
#48740=CARTESIAN_POINT('',(-1.10653577764992,-0.05953,-0.196295654879793));
#48741=CARTESIAN_POINT('Origin',(0.,-0.05953,0.));
#48742=CARTESIAN_POINT('',(-0.843383895613249,-0.05953,-0.742736168477219));
#48743=CARTESIAN_POINT('Ctrl Pts',(-1.10653577764992,-0.0595300000000001,
-0.196295654879792));
#48744=CARTESIAN_POINT('Ctrl Pts',(-1.10595102243643,-0.0762225747374255,
-0.199591971170104));
#48745=CARTESIAN_POINT('Ctrl Pts',(-1.10509821673782,-0.0928409665394228,
-0.204327142733962));
#48746=CARTESIAN_POINT('Ctrl Pts',(-1.10139388218929,-0.144299303100741,
-0.22376314604679));
#48747=CARTESIAN_POINT('Ctrl Pts',(-1.09728268713976,-0.177024326825049,
-0.243890930799338));
#48748=CARTESIAN_POINT('Ctrl Pts',(-1.08664560412098,-0.227269801620063,
-0.287406530683753));
#48749=CARTESIAN_POINT('Ctrl Pts',(-1.0788165083757,-0.251265615809407,
-0.316022600643821));
#48750=CARTESIAN_POINT('Ctrl Pts',(-1.06356957703048,-0.279889827963178,
-0.363699428370918));
#48751=CARTESIAN_POINT('Ctrl Pts',(-1.05494634094458,-0.290879136862659,
-0.388295406390235));
#48752=CARTESIAN_POINT('Ctrl Pts',(-1.03504317708586,-0.305251990234488,
-0.438600874831839));
#48753=CARTESIAN_POINT('Ctrl Pts',(-1.02374168767024,-0.308638795020976,
-0.46430090015576));
#48754=CARTESIAN_POINT('Ctrl Pts',(-1.00129756308006,-0.308638795020976,
-0.510906605094603));
#48755=CARTESIAN_POINT('Ctrl Pts',(-0.988250837578047,-0.305251990234488,
-0.535766169015486));
#48756=CARTESIAN_POINT('Ctrl Pts',(-0.961329858300736,-0.290879136862659,
-0.582692035672022));
#48757=CARTESIAN_POINT('Ctrl Pts',(-0.947476448101718,-0.279889827963178,
-0.604769294586516));
#48758=CARTESIAN_POINT('Ctrl Pts',(-0.919707509403859,-0.251265615809407,
-0.646415841396062));
#48759=CARTESIAN_POINT('Ctrl Pts',(-0.902215926359523,-0.227269801620064,
-0.670378702718353));
#48760=CARTESIAN_POINT('Ctrl Pts',(-0.87482617317514,-0.177024326825049,
-0.705826641853758));
#48761=CARTESIAN_POINT('Ctrl Pts',(-0.861652925570091,-0.144299303100741,
-0.721590372101268));
#48762=CARTESIAN_POINT('Ctrl Pts',(-0.848766861100456,-0.0928409665394229,
-0.736604687327351));
#48763=CARTESIAN_POINT('Ctrl Pts',(-0.84559647055299,-0.0762225747374255,
-0.740223768851063));
#48764=CARTESIAN_POINT('Ctrl Pts',(-0.843383895613249,-0.0595300000000001,
-0.742736168477219));
#48765=CARTESIAN_POINT('',(-0.536443649899847,-0.05953,-0.987512846410683));
#48766=CARTESIAN_POINT('Origin',(0.,-0.05953,0.));
#48767=CARTESIAN_POINT('',(0.0548532617164172,-0.05953,-1.12247250791415));
#48768=CARTESIAN_POINT('Ctrl Pts',(-0.536443649899848,-0.0595300000000001,
-0.987512846410683));
#48769=CARTESIAN_POINT('Ctrl Pts',(-0.533501897135712,-0.0762225747374254,
-0.989110885965947));
#48770=CARTESIAN_POINT('Ctrl Pts',(-0.529268075276156,-0.0928409665394227,
-0.991396466802469));
#48771=CARTESIAN_POINT('Ctrl Pts',(-0.511762781179147,-0.144299303100741,
-1.00061845128527));
#48772=CARTESIAN_POINT('Ctrl Pts',(-0.493462957200432,-0.177024326825049,
-1.0099536580922));
#48773=CARTESIAN_POINT('Ctrl Pts',(-0.45280897844858,-0.227269801620063,
-1.02876878445619));
#48774=CARTESIAN_POINT('Ctrl Pts',(-0.425554672694337,-0.251265615809407,
-1.04048957871266));
#48775=CARTESIAN_POINT('Ctrl Pts',(-0.3787731215897,-0.279889827963178,
-1.05829506364875));
#48776=CARTESIAN_POINT('Ctrl Pts',(-0.354166711873529,-0.290879136862659,
-1.06688848765783));
#48777=CARTESIAN_POINT('Ctrl Pts',(-0.302426893214944,-0.305251990234488,
-1.08269251410343));
#48778=CARTESIAN_POINT('Ctrl Pts',(-0.275287440920027,-0.308638795020976,
-1.0898803575765));
#48779=CARTESIAN_POINT('Ctrl Pts',(-0.224855950742601,-0.308638795020976,
-1.10139101611326));
#48780=CARTESIAN_POINT('Ctrl Pts',(-0.19728546073067,-0.305251990234488,
-1.10669035995599));
#48781=CARTESIAN_POINT('Ctrl Pts',(-0.143812384801039,-0.290879136862659,
-1.11490049012186));
#48782=CARTESIAN_POINT('Ctrl Pts',(-0.117914228755037,-0.279889827963178,
-1.1178344036749));
#48783=CARTESIAN_POINT('Ctrl Pts',(-0.0680399972366989,-0.251265615809407,
-1.12208997038458));
#48784=CARTESIAN_POINT('Ctrl Pts',(-0.0383992541984084,-0.227269801620063,
-1.12335509974011));
#48785=CARTESIAN_POINT('Ctrl Pts',(0.00639229239215326,-0.177024326825049,
-1.12404235695137));
#48786=CARTESIAN_POINT('Ctrl Pts',(0.0269302585198977,-0.144299303100741,
-1.12357162229597));
#48787=CARTESIAN_POINT('Ctrl Pts',(0.04670325263426,-0.0928409665394228,
-1.12285816383385));
#48788=CARTESIAN_POINT('Ctrl Pts',(0.0515094706813703,-0.0762225747374255,
-1.12263591311425));
#48789=CARTESIAN_POINT('Ctrl Pts',(0.0548532617164176,-0.0595300000000001,
-1.12247250791414));
#48790=CARTESIAN_POINT('',(0.437601487681057,-0.05953,-1.03511272300331));
#48791=CARTESIAN_POINT('Origin',(0.,-0.05953,0.));
#48792=CARTESIAN_POINT('',(0.911784794170997,-0.05953,-0.656964154625313));
#48793=CARTESIAN_POINT('Ctrl Pts',(0.437601487681056,-0.0595300000000001,
-1.03511272300331));
#48794=CARTESIAN_POINT('Ctrl Pts',(0.440685038163619,-0.0762225747374255,
-1.03380912944435));
#48795=CARTESIAN_POINT('Ctrl Pts',(0.445111721969657,-0.0928409665394228,
-1.03192403056628));
#48796=CARTESIAN_POINT('Ctrl Pts',(0.463236132117164,-0.144299303100741,
-1.0239876538093));
#48797=CARTESIAN_POINT('Ctrl Pts',(0.481944444320713,-0.177024326825049,
-1.01550068154148));
#48798=CARTESIAN_POINT('Ctrl Pts',(0.522002043615455,-0.227269801620064,
-0.995447160474328));
#48799=CARTESIAN_POINT('Ctrl Pts',(0.548158511259203,-0.251265615809407,
-0.981446681891443));
#48800=CARTESIAN_POINT('Ctrl Pts',(0.591247219971725,-0.279889827963178,
-0.955972930713954));
#48801=CARTESIAN_POINT('Ctrl Pts',(0.613307674922609,-0.290879136862659,
-0.942092777160053));
#48802=CARTESIAN_POINT('Ctrl Pts',(0.657923009631182,-0.305251990234487,
-0.91149460735272));
#48803=CARTESIAN_POINT('Ctrl Pts',(0.680463863683393,-0.308638795020976,
-0.894757676234429));
#48804=CARTESIAN_POINT('Ctrl Pts',(0.720906778729542,-0.308638795020976,
-0.862505527716294));
#48805=CARTESIAN_POINT('Ctrl Pts',(0.742239891936899,-0.305251990234488,
-0.844254137480381));
#48806=CARTESIAN_POINT('Ctrl Pts',(0.781998747691872,-0.290879136862659,
-0.80756613568454));
#48807=CARTESIAN_POINT('Ctrl Pts',(0.800439809856112,-0.279889827963178,
-0.789147407129765));
#48808=CARTESIAN_POINT('Ctrl Pts',(0.834863020612702,-0.251265615809407,
-0.752807465209441));
#48809=CARTESIAN_POINT('Ctrl Pts',(0.854332839576145,-0.227269801620064,
-0.73042219438957));
#48810=CARTESIAN_POINT('Ctrl Pts',(0.882797231409153,-0.177024326825049,
-0.695831250979106));
#48811=CARTESIAN_POINT('Ctrl Pts',(0.895234408667242,-0.144299303100741,
-0.679480524217551));
#48812=CARTESIAN_POINT('Ctrl Pts',(0.907004864562642,-0.0928409665394228,
-0.663576540841106));
#48813=CARTESIAN_POINT('Ctrl Pts',(0.909827729890942,-0.0762225747374256,
-0.659680317203144));
#48814=CARTESIAN_POINT('Ctrl Pts',(0.911784794170998,-0.0595300000000001,
-0.656964154625312));
#48815=CARTESIAN_POINT('',(1.08212377959455,-0.05953,-0.303251606722892));
#48816=CARTESIAN_POINT('Origin',(0.,-0.05953,0.));
#48817=CARTESIAN_POINT('',(1.08212377959455,-0.05953,0.303251606722892));
#48818=CARTESIAN_POINT('Ctrl Pts',(1.08212377959455,-0.0595300000000001,
-0.303251606722892));
#48819=CARTESIAN_POINT('Ctrl Pts',(1.0830271513892,-0.0762225747374255,
-0.300028012588062));
#48820=CARTESIAN_POINT('Ctrl Pts',(1.08431331394788,-0.0928409665394228,
-0.2953917518996));
#48821=CARTESIAN_POINT('Ctrl Pts',(1.08940878963422,-0.144299303100741,
-0.276273267473431));
#48822=CARTESIAN_POINT('Ctrl Pts',(1.09443784939331,-0.177024326825049,
-0.256354979351213));
#48823=CARTESIAN_POINT('Ctrl Pts',(1.10373487993589,-0.227269801620064,
-0.212533521233765));
#48824=CARTESIAN_POINT('Ctrl Pts',(1.10909715583869,-0.251265615809407,
-0.183354415742157));
#48825=CARTESIAN_POINT('Ctrl Pts',(1.1160463456491,-0.279889827963178,-0.133783682657561));
#48826=CARTESIAN_POINT('Ctrl Pts',(1.11894887330541,-0.290879136862659,
-0.107881990270302));
#48827=CARTESIAN_POINT('Ctrl Pts',(1.12284346704144,-0.305251990234488,
-0.0539226701638766));
#48828=CARTESIAN_POINT('Ctrl Pts',(1.123812,-0.308638795020976,-0.025864214957475));
#48829=CARTESIAN_POINT('Ctrl Pts',(1.123812,-0.308638795020976,0.025864214957475));
#48830=CARTESIAN_POINT('Ctrl Pts',(1.12284346704144,-0.305251990234488,
0.0539226701638766));
#48831=CARTESIAN_POINT('Ctrl Pts',(1.11894887330541,-0.290879136862659,
0.107881990270302));
#48832=CARTESIAN_POINT('Ctrl Pts',(1.1160463456491,-0.279889827963178,0.133783682657561));
#48833=CARTESIAN_POINT('Ctrl Pts',(1.10909715583869,-0.251265615809407,
0.183354415742157));
#48834=CARTESIAN_POINT('Ctrl Pts',(1.10373487993589,-0.227269801620064,
0.212533521233765));
#48835=CARTESIAN_POINT('Ctrl Pts',(1.09443784939331,-0.177024326825049,
0.256354979351213));
#48836=CARTESIAN_POINT('Ctrl Pts',(1.08940878963422,-0.144299303100741,
0.276273267473431));
#48837=CARTESIAN_POINT('Ctrl Pts',(1.08431331394788,-0.0928409665394228,
0.2953917518996));
#48838=CARTESIAN_POINT('Ctrl Pts',(1.0830271513892,-0.0762225747374255,
0.300028012588062));
#48839=CARTESIAN_POINT('Ctrl Pts',(1.08212377959455,-0.0595300000000001,
0.303251606722892));
#48840=CARTESIAN_POINT('Origin',(0.,-0.05953,0.));
#48841=CARTESIAN_POINT('Origin',(0.,-0.05953,0.));
#48842=CARTESIAN_POINT('',(0.0589974094846122,-0.05953,1.07456964270265));
#48843=CARTESIAN_POINT('Origin',(0.,-0.05953,0.));
#48844=CARTESIAN_POINT('Origin',(-0.244773027351946,-0.05953,1.07242070340001));
#48845=CARTESIAN_POINT('Origin',(-0.244773027351946,0.,1.07242070340001));
#48846=CARTESIAN_POINT('',(-0.519393123750572,-0.05953,0.942555777842682));
#48847=CARTESIAN_POINT('Ctrl Pts',(-0.519393123750572,-0.05953,0.942555777842682));
#48848=CARTESIAN_POINT('Ctrl Pts',(-0.513714466572041,-0.0925528133349865,
0.945684988399766));
#48849=CARTESIAN_POINT('Ctrl Pts',(-0.503136848051455,-0.124911173756694,
0.951483858396181));
#48850=CARTESIAN_POINT('Ctrl Pts',(-0.47593627990192,-0.177924977804098,
0.965323333309091));
#48851=CARTESIAN_POINT('Ctrl Pts',(-0.460931856495794,-0.199697230012983,
0.972669835243841));
#48852=CARTESIAN_POINT('Ctrl Pts',(-0.426157505475872,-0.237895043532788,
0.988400002689705));
#48853=CARTESIAN_POINT('Ctrl Pts',(-0.406380688682952,-0.254319232363049,
0.996771768218699));
#48854=CARTESIAN_POINT('Ctrl Pts',(-0.364750145543744,-0.28018331644634,
1.01272583306292));
#48855=CARTESIAN_POINT('Ctrl Pts',(-0.340838910881557,-0.29104845371857,
1.02112815447116));
#48856=CARTESIAN_POINT('Ctrl Pts',(-0.290495481564827,-0.30527573347708,
1.036574285215));
#48857=CARTESIAN_POINT('Ctrl Pts',(-0.264056468041074,-0.308638795020976,
1.04359501395068));
#48858=CARTESIAN_POINT('Ctrl Pts',(-0.214892249704082,-0.308638795020976,
1.05481642595959));
#48859=CARTESIAN_POINT('Ctrl Pts',(-0.188025341585962,-0.30527573347708,
1.05996242598502));
#48860=CARTESIAN_POINT('Ctrl Pts',(-0.135965654106109,-0.29104845371857,
1.06788913840721));
#48861=CARTESIAN_POINT('Ctrl Pts',(-0.110776745452494,-0.28018331644634,
1.07069360430242));
#48862=CARTESIAN_POINT('Ctrl Pts',(-0.0663467128214646,-0.254319232363049,
1.07438230428002));
#48863=CARTESIAN_POINT('Ctrl Pts',(-0.0448960436540983,-0.237895043532788,
1.07542044338697));
#48864=CARTESIAN_POINT('Ctrl Pts',(-0.00674037211528124,-0.199697230012983,
1.07633607767727));
#48865=CARTESIAN_POINT('Ctrl Pts',(0.00996567398334777,-0.177924977804098,
1.07622728347683));
#48866=CARTESIAN_POINT('Ctrl Pts',(0.0404772621979741,-0.124911173756694,
1.07556023164702));
#48867=CARTESIAN_POINT('Ctrl Pts',(0.0525234025782719,-0.0925528133349865,
1.07492508698591));
#48868=CARTESIAN_POINT('Ctrl Pts',(0.0589974094846124,-0.05953,1.07456964270265));
#48869=CARTESIAN_POINT('Origin',(-0.244773027351946,-0.05953,1.07242070340001));
#48870=CARTESIAN_POINT('Origin',(0.,-0.05953,0.));
#48871=CARTESIAN_POINT('',(-0.803348093619616,-0.05953,0.716109245731214));
#48872=CARTESIAN_POINT('Origin',(0.,-0.05953,0.));
#48873=CARTESIAN_POINT('Origin',(-0.991065754692661,-0.05953,0.477272113029314));
#48874=CARTESIAN_POINT('Origin',(-0.991065754692661,0.,0.477272113029314));
#48875=CARTESIAN_POINT('',(-1.06075609691358,-0.05953,0.181596019242328));
#48876=CARTESIAN_POINT('Ctrl Pts',(-1.06075609691358,-0.05953,0.181596019242328));
#48877=CARTESIAN_POINT('Ctrl Pts',(-1.05966202740332,-0.0925528133349865,
0.187986803072856));
#48878=CARTESIAN_POINT('Ctrl Pts',(-1.05760072925372,-0.124911173756694,
0.199872254546857));
#48879=CARTESIAN_POINT('Ctrl Pts',(-1.05146158959546,-0.177924977804098,
0.22976728653846));
#48880=CARTESIAN_POINT('Ctrl Pts',(-1.04785021111757,-0.199697230012983,
0.246078686169301));
#48881=CARTESIAN_POINT('Ctrl Pts',(-1.03846709802406,-0.237895043532788,
0.283073967563097));
#48882=CARTESIAN_POINT('Ctrl Pts',(-1.03268176429485,-0.254319232363049,
0.303755815985685));
#48883=CARTESIAN_POINT('Ctrl Pts',(-1.01919893537026,-0.28018331644634,
0.346251081972725));
#48884=CARTESIAN_POINT('Ctrl Pts',(-1.01085972381132,-0.29104845371857,
0.370184399726282));
#48885=CARTESIAN_POINT('Ctrl Pts',(-0.99154738033959,-0.30527573347708,
0.419174982698463));
#48886=CARTESIAN_POINT('Ctrl Pts',(-0.980551951791748,-0.308638795020976,
0.444223188605045));
#48887=CARTESIAN_POINT('Ctrl Pts',(-0.958671816228589,-0.308638795020976,
0.489657758261848));
#48888=CARTESIAN_POINT('Ctrl Pts',(-0.945943877838127,-0.30527573347708,
0.51387163140139));
#48889=CARTESIAN_POINT('Ctrl Pts',(-0.91968254693063,-0.29104845371857,
0.559515758398093));
#48890=CARTESIAN_POINT('Ctrl Pts',(-0.906170138993533,-0.28018331644634,
0.580957796077825));
#48891=CARTESIAN_POINT('Ctrl Pts',(-0.8813524085237,-0.254319232363049,
0.617994461173994));
#48892=CARTESIAN_POINT('Ctrl Pts',(-0.868789784891799,-0.237895043532788,
0.635412538795143));
#48893=CARTESIAN_POINT('Ctrl Pts',(-0.845715984518854,-0.199697230012983,
0.66581473268113));
#48894=CARTESIAN_POINT('Ctrl Pts',(-0.835214876415962,-0.177924977804098,
0.678808213394124));
#48895=CARTESIAN_POINT('Ctrl Pts',(-0.815669690204649,-0.124911173756694,
0.702247233627224));
#48896=CARTESIAN_POINT('Ctrl Pts',(-0.807662468433796,-0.0925528133349865,
0.711269279199861));
#48897=CARTESIAN_POINT('Ctrl Pts',(-0.803348093619616,-0.05953,0.716109245731214));
#48898=CARTESIAN_POINT('Origin',(-0.991065754692661,-0.05953,0.477272113029314));
#48899=CARTESIAN_POINT('Origin',(0.,-0.05953,0.));
#48900=CARTESIAN_POINT('',(-1.076188,-0.05953,1.31795018948079E-16));
#48901=CARTESIAN_POINT('Origin',(0.,-0.05953,0.));
#48902=CARTESIAN_POINT('',(-1.06075609691358,-0.05953,-0.181596019242328));
#48903=CARTESIAN_POINT('Origin',(0.,-0.05953,0.));
#48904=CARTESIAN_POINT('Origin',(-0.991065754692661,-0.05953,-0.477272113029314));
#48905=CARTESIAN_POINT('Origin',(-0.991065754692661,0.,-0.477272113029314));
#48906=CARTESIAN_POINT('',(-0.803348093619616,-0.05953,-0.716109245731215));
#48907=CARTESIAN_POINT('Ctrl Pts',(-0.803348093619616,-0.05953,-0.716109245731215));
#48908=CARTESIAN_POINT('Ctrl Pts',(-0.807662468433795,-0.0925528133349865,
-0.711269279199862));
#48909=CARTESIAN_POINT('Ctrl Pts',(-0.815669690204649,-0.124911173756694,
-0.702247233627224));
#48910=CARTESIAN_POINT('Ctrl Pts',(-0.835214876415962,-0.177924977804098,
-0.678808213394124));
#48911=CARTESIAN_POINT('Ctrl Pts',(-0.845715984518854,-0.199697230012983,
-0.66581473268113));
#48912=CARTESIAN_POINT('Ctrl Pts',(-0.868789784891799,-0.237895043532788,
-0.635412538795143));
#48913=CARTESIAN_POINT('Ctrl Pts',(-0.8813524085237,-0.254319232363049,
-0.617994461173994));
#48914=CARTESIAN_POINT('Ctrl Pts',(-0.906170138993533,-0.28018331644634,
-0.580957796077826));
#48915=CARTESIAN_POINT('Ctrl Pts',(-0.91968254693063,-0.29104845371857,
-0.559515758398093));
#48916=CARTESIAN_POINT('Ctrl Pts',(-0.945943877838127,-0.30527573347708,
-0.51387163140139));
#48917=CARTESIAN_POINT('Ctrl Pts',(-0.958671816228589,-0.308638795020976,
-0.489657758261848));
#48918=CARTESIAN_POINT('Ctrl Pts',(-0.980551951791748,-0.308638795020976,
-0.444223188605045));
#48919=CARTESIAN_POINT('Ctrl Pts',(-0.99154738033959,-0.30527573347708,
-0.419174982698463));
#48920=CARTESIAN_POINT('Ctrl Pts',(-1.01085972381132,-0.29104845371857,
-0.370184399726282));
#48921=CARTESIAN_POINT('Ctrl Pts',(-1.01919893537026,-0.28018331644634,
-0.346251081972725));
#48922=CARTESIAN_POINT('Ctrl Pts',(-1.03268176429485,-0.254319232363049,
-0.303755815985685));
#48923=CARTESIAN_POINT('Ctrl Pts',(-1.03846709802406,-0.237895043532788,
-0.283073967563097));
#48924=CARTESIAN_POINT('Ctrl Pts',(-1.04785021111757,-0.199697230012983,
-0.246078686169302));
#48925=CARTESIAN_POINT('Ctrl Pts',(-1.05146158959546,-0.177924977804098,
-0.229767286538461));
#48926=CARTESIAN_POINT('Ctrl Pts',(-1.05760072925372,-0.124911173756694,
-0.199872254546858));
#48927=CARTESIAN_POINT('Ctrl Pts',(-1.05966202740332,-0.0925528133349864,
-0.187986803072857));
#48928=CARTESIAN_POINT('Ctrl Pts',(-1.06075609691358,-0.05953,-0.181596019242328));
#48929=CARTESIAN_POINT('Origin',(-0.991065754692661,-0.05953,-0.477272113029314));
#48930=CARTESIAN_POINT('Origin',(0.,-0.05953,0.));
#48931=CARTESIAN_POINT('',(-0.519393123750572,-0.05953,-0.942555777842682));
#48932=CARTESIAN_POINT('Origin',(0.,-0.05953,0.));
#48933=CARTESIAN_POINT('Origin',(-0.244773027351946,-0.05953,-1.07242070340001));
#48934=CARTESIAN_POINT('Origin',(-0.244773027351946,0.,-1.07242070340001));
#48935=CARTESIAN_POINT('',(0.0589974094846125,-0.05953,-1.07456964270265));
#48936=CARTESIAN_POINT('Ctrl Pts',(0.0589974094846127,-0.05953,-1.07456964270265));
#48937=CARTESIAN_POINT('Ctrl Pts',(0.0525234025782722,-0.0925528133349865,
-1.07492508698591));
#48938=CARTESIAN_POINT('Ctrl Pts',(0.0404772621979744,-0.124911173756694,
-1.07556023164702));
#48939=CARTESIAN_POINT('Ctrl Pts',(0.0099656739833481,-0.177924977804098,
-1.07622728347683));
#48940=CARTESIAN_POINT('Ctrl Pts',(-0.00674037211528096,-0.199697230012983,
-1.07633607767727));
#48941=CARTESIAN_POINT('Ctrl Pts',(-0.044896043654098,-0.237895043532788,
-1.07542044338697));
#48942=CARTESIAN_POINT('Ctrl Pts',(-0.0663467128214644,-0.254319232363049,
-1.07438230428002));
#48943=CARTESIAN_POINT('Ctrl Pts',(-0.110776745452493,-0.28018331644634,
-1.07069360430242));
#48944=CARTESIAN_POINT('Ctrl Pts',(-0.135965654106109,-0.29104845371857,
-1.06788913840721));
#48945=CARTESIAN_POINT('Ctrl Pts',(-0.188025341585962,-0.30527573347708,
-1.05996242598502));
#48946=CARTESIAN_POINT('Ctrl Pts',(-0.214892249704082,-0.308638795020976,
-1.05481642595959));
#48947=CARTESIAN_POINT('Ctrl Pts',(-0.264056468041074,-0.308638795020976,
-1.04359501395068));
#48948=CARTESIAN_POINT('Ctrl Pts',(-0.290495481564827,-0.30527573347708,
-1.036574285215));
#48949=CARTESIAN_POINT('Ctrl Pts',(-0.340838910881557,-0.291048453718569,
-1.02112815447116));
#48950=CARTESIAN_POINT('Ctrl Pts',(-0.364750145543744,-0.28018331644634,
-1.01272583306292));
#48951=CARTESIAN_POINT('Ctrl Pts',(-0.406380688682952,-0.254319232363049,
-0.996771768218699));
#48952=CARTESIAN_POINT('Ctrl Pts',(-0.426157505475872,-0.237895043532788,
-0.988400002689705));
#48953=CARTESIAN_POINT('Ctrl Pts',(-0.460931856495794,-0.199697230012983,
-0.972669835243841));
#48954=CARTESIAN_POINT('Ctrl Pts',(-0.475936279901919,-0.177924977804098,
-0.965323333309091));
#48955=CARTESIAN_POINT('Ctrl Pts',(-0.503136848051454,-0.124911173756694,
-0.951483858396181));
#48956=CARTESIAN_POINT('Ctrl Pts',(-0.513714466572041,-0.0925528133349865,
-0.945684988399766));
#48957=CARTESIAN_POINT('Ctrl Pts',(-0.519393123750572,-0.05953,-0.942555777842682));
#48958=CARTESIAN_POINT('Origin',(-0.244773027351946,-0.05953,-1.07242070340001));
#48959=CARTESIAN_POINT('Origin',(0.,-0.05953,0.));
#48960=CARTESIAN_POINT('',(0.413083465285518,-0.05953,-0.993751811093549));
#48961=CARTESIAN_POINT('Origin',(0.,-0.05953,0.));
#48962=CARTESIAN_POINT('Origin',(0.685838782044607,-0.05953,-0.860014630714833));
#48963=CARTESIAN_POINT('Origin',(0.685838782044607,0.,-0.860014630714833));
#48964=CARTESIAN_POINT('',(0.876916659919095,-0.05953,-0.623857181492959));
#48965=CARTESIAN_POINT('Ctrl Pts',(0.876916659919095,-0.05953,-0.623857181492958));
#48966=CARTESIAN_POINT('Ctrl Pts',(0.873158080166742,-0.0925528133349865,
-0.62914037979579));
#48967=CARTESIAN_POINT('Ctrl Pts',(0.866144010579847,-0.124911173756694,
-0.638954437806245));
#48968=CARTESIAN_POINT('Ctrl Pts',(0.847641868610495,-0.177924977804098,
-0.663225258065736));
#48969=CARTESIAN_POINT('Ctrl Pts',(0.837310877969633,-0.199697230012983,
-0.676354402927683));
#48970=CARTESIAN_POINT('Ctrl Pts',(0.81280533416753,-0.237895043532788,
-0.705614819529209));
#48971=CARTESIAN_POINT('Ctrl Pts',(0.798619410861634,-0.254319232363049,
-0.721738358858166));
#48972=CARTESIAN_POINT('Ctrl Pts',(0.768033796848072,-0.28018331644634,
-0.754175290318038));
#48973=CARTESIAN_POINT('Ctrl Pts',(0.750136149454208,-0.29104845371857,
-0.772120216227122));
#48974=CARTESIAN_POINT('Ctrl Pts',(0.711480111898423,-0.30527573347708,
-0.807879894508811));
#48975=CARTESIAN_POINT('Ctrl Pts',(0.690705563850638,-0.308638795020976,
-0.825676810575913));
#48976=CARTESIAN_POINT('Ctrl Pts',(0.651278921914856,-0.308638795020976,
-0.857118508332695));
#48977=CARTESIAN_POINT('Ctrl Pts',(0.629305439856167,-0.30527573347708,
-0.873412008702649));
#48978=CARTESIAN_POINT('Ctrl Pts',(0.585840553788742,-0.29104845371857,
-0.903141581680914));
#48979=CARTESIAN_POINT('Ctrl Pts',(0.564362943424239,-0.28018331644634,
-0.916597376014514));
#48980=CARTESIAN_POINT('Ctrl Pts',(0.525933334162556,-0.254319232363049,
-0.939198248544427));
#48981=CARTESIAN_POINT('Ctrl Pts',(0.507057380724533,-0.237895043532788,
-0.949440676105255));
#48982=CARTESIAN_POINT('Ctrl Pts',(0.473077587363686,-0.199697230012983,
-0.966820759530997));
#48983=CARTESIAN_POINT('Ctrl Pts',(0.457978755888596,-0.177924977804098,
-0.973971221090534));
#48984=CARTESIAN_POINT('Ctrl Pts',(0.430199341854858,-0.124911173756694,
-0.986608710139579));
#48985=CARTESIAN_POINT('Ctrl Pts',(0.419070565453384,-0.0925528133349865,
-0.991263089003441));
#48986=CARTESIAN_POINT('Ctrl Pts',(0.413083465285518,-0.05953,-0.993751811093549));
#48987=CARTESIAN_POINT('Origin',(0.685838782044607,-0.05953,-0.860014630714833));
#48988=CARTESIAN_POINT('Origin',(0.,-0.208355,0.));
#48989=CARTESIAN_POINT('',(-1.076188,-0.35718,1.31795018948079E-16));
#48990=CARTESIAN_POINT('Origin',(0.,-0.35718,0.));
#48991=CARTESIAN_POINT('',(-1.076188,-0.208355,1.31795018948079E-16));
#48992=CARTESIAN_POINT('',(1.03449977959455,-0.05953,0.296632461748266));
#48993=CARTESIAN_POINT('Origin',(0.,-0.05953,0.));
#48994=CARTESIAN_POINT('',(1.03449977959455,-0.05953,-0.296632461748266));
#48995=CARTESIAN_POINT('Ctrl Pts',(1.03449977959455,-0.05953,0.296632461748267));
#48996=CARTESIAN_POINT('Ctrl Pts',(1.03628691421076,-0.0925528133349865,
0.290399865505497));
#48997=CARTESIAN_POINT('Ctrl Pts',(1.03958665287714,-0.124911173756694,
0.278797079997872));
#48998=CARTESIAN_POINT('Ctrl Pts',(1.0470264474309,-0.177924977804098,0.249198913998601));
#48999=CARTESIAN_POINT('Ctrl Pts',(1.05084995891418,-0.199697230012983,
0.232935932341942));
#49000=CARTESIAN_POINT('Ctrl Pts',(1.05844771715377,-0.237895043532788,
0.195533155353269));
#49001=CARTESIAN_POINT('Ctrl Pts',(1.06220882929878,-0.254319232363049,
0.17438929156337));
#49002=CARTESIAN_POINT('Ctrl Pts',(1.06849922508772,-0.28018331644634,0.130252399648131));
#49003=CARTESIAN_POINT('Ctrl Pts',(1.07137013248666,-0.29104845371857,0.105070977154072));
#49004=CARTESIAN_POINT('Ctrl Pts',(1.07522652957392,-0.30527573347708,0.0525526752791107));
#49005=CARTESIAN_POINT('Ctrl Pts',(1.076188,-0.308638795020976,0.025214283908933));
#49006=CARTESIAN_POINT('Ctrl Pts',(1.076188,-0.308638795020976,-0.025214283908933));
#49007=CARTESIAN_POINT('Ctrl Pts',(1.07522652957392,-0.30527573347708,-0.0525526752791107));
#49008=CARTESIAN_POINT('Ctrl Pts',(1.07137013248666,-0.29104845371857,-0.105070977154072));
#49009=CARTESIAN_POINT('Ctrl Pts',(1.06849922508772,-0.28018331644634,-0.130252399648131));
#49010=CARTESIAN_POINT('Ctrl Pts',(1.06220882929878,-0.254319232363049,
-0.17438929156337));
#49011=CARTESIAN_POINT('Ctrl Pts',(1.05844771715377,-0.237895043532788,
-0.195533155353269));
#49012=CARTESIAN_POINT('Ctrl Pts',(1.05084995891418,-0.199697230012983,
-0.232935932341942));
#49013=CARTESIAN_POINT('Ctrl Pts',(1.0470264474309,-0.177924977804098,-0.249198913998601));
#49014=CARTESIAN_POINT('Ctrl Pts',(1.03958665287714,-0.124911173756694,
-0.278797079997872));
#49015=CARTESIAN_POINT('Ctrl Pts',(1.03628691421076,-0.0925528133349865,
-0.290399865505497));
#49016=CARTESIAN_POINT('Ctrl Pts',(1.03449977959455,-0.05953,-0.296632461748267));
#49017=CARTESIAN_POINT('Origin',(0.,-0.05953,0.));
#49018=CARTESIAN_POINT('Origin',(0.,-0.05953,0.));
#49019=CARTESIAN_POINT('Origin',(1.1,-0.05953,0.));
#49020=CARTESIAN_POINT('Origin',(1.1,0.,0.));
#49021=CARTESIAN_POINT('Origin',(1.1,-0.05953,0.));
#49022=CARTESIAN_POINT('Origin',(0.,-0.35718,0.));
#49023=CARTESIAN_POINT('Origin',(0.,-0.05953,0.));
#62852=UNCERTAINTY_MEASURE_WITH_UNIT(LENGTH_MEASURE(0.001),#62985,
'DISTANCE_ACCURACY_VALUE',
'Maximum model space distance between geometric entities at asserted c
onnectivities');
#62885=UNCERTAINTY_MEASURE_WITH_UNIT(LENGTH_MEASURE(0.001),#62985,
'DISTANCE_ACCURACY_VALUE',
'Maximum model space distance between geometric entities at asserted c
onnectivities');
#62951=(
GEOMETRIC_REPRESENTATION_CONTEXT(3)
GLOBAL_UNCERTAINTY_ASSIGNED_CONTEXT((#62852))
GLOBAL_UNIT_ASSIGNED_CONTEXT((#62985,#62987,#62988))
REPRESENTATION_CONTEXT('','3D')
);
#62984=(
GEOMETRIC_REPRESENTATION_CONTEXT(3)
GLOBAL_UNCERTAINTY_ASSIGNED_CONTEXT((#62885))
GLOBAL_UNIT_ASSIGNED_CONTEXT((#62985,#62987,#62988))
REPRESENTATION_CONTEXT('','3D')
);
#62985=(
LENGTH_UNIT()
NAMED_UNIT(*)
SI_UNIT(.CENTI.,.METRE.)
);
#62987=(
NAMED_UNIT(*)
PLANE_ANGLE_UNIT()
SI_UNIT($,.RADIAN.)
);
#62988=(
NAMED_UNIT(*)
SI_UNIT($,.STERADIAN.)
SOLID_ANGLE_UNIT()
);
#63054=SHAPE_DEFINITION_REPRESENTATION(#63232,#63414);
#63232=PRODUCT_DEFINITION_SHAPE('',$,#63513);
#63414=SHAPE_REPRESENTATION('',(#25586),#62951);
#63447=PRODUCT_DEFINITION_CONTEXT('part definition',#63743,'design');
#63513=PRODUCT_DEFINITION('Cage (2)','Cage (2)',#63611,#63447);
#63611=PRODUCT_DEFINITION_FORMATION('',$,#63810);
#63743=APPLICATION_CONTEXT(
'Core Data for Automotive Mechanical Design Process');
#63744=PRODUCT_CONTEXT('part definition',#63743,'mechanical');
#63810=PRODUCT('Cage (2)','Cage (2)','Cage (2)',(#63744));
#63906=COLOUR_RGB('Grey',0.48,0.52,0.57);
#63907=FILL_AREA_STYLE_COLOUR('',#63906);
#63908=FILL_AREA_STYLE('',(#63907));
#63909=SURFACE_STYLE_FILL_AREA(#63908);
#63910=SURFACE_SIDE_STYLE('',(#63909));
#63911=SURFACE_STYLE_USAGE(.BOTH.,#63910);
#63912=PRESENTATION_STYLE_ASSIGNMENT((#63911));
ENDSEC;
END-ISO-10303-21;
